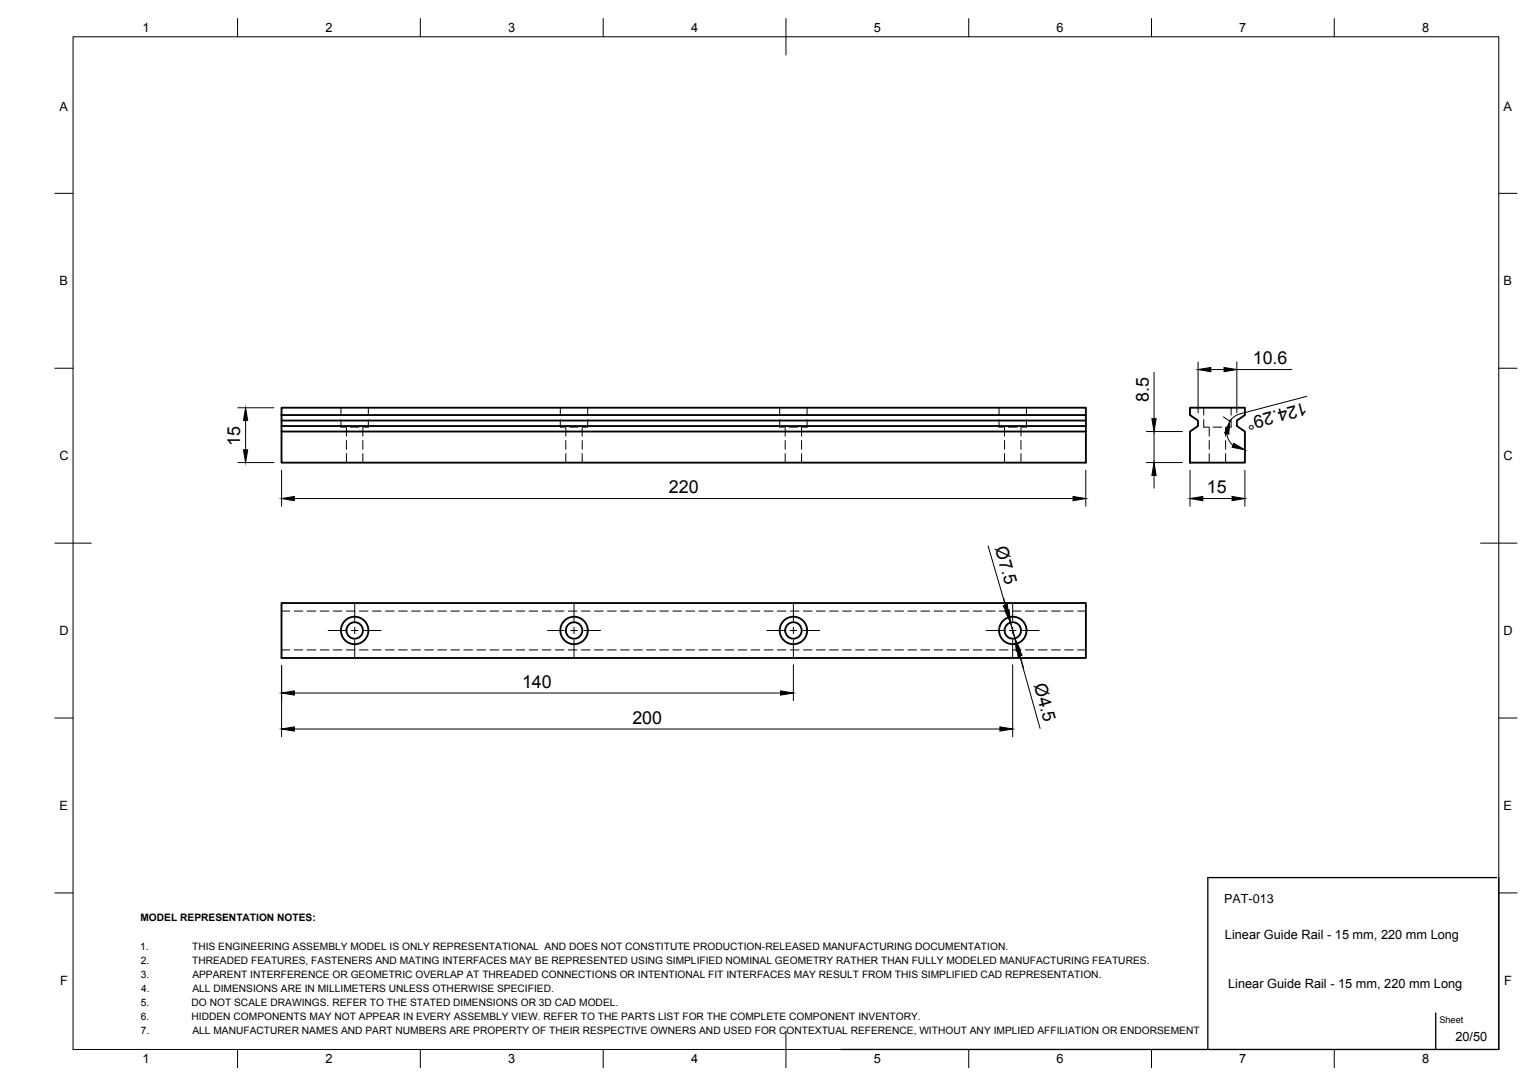
ISO-10303-21;
HEADER;
/* Generated by software containing ST-Developer
 * from STEP Tools, Inc. (www.steptools.com) 
 */

FILE_DESCRIPTION(
/* description */ ('Belt-driven linear axis on 2020 extrusion'),
/* implementation_level */ '2;1');

FILE_NAME(
/* name */ 'Linear Guide Rail - 15 mm, 220 mm Long.step',
/* time_stamp */ '2026-10-28T03:26:09-07:00',
/* author */ (''),
/* organization */ (''),
/* preprocessor_version */ 'ST-DEVELOPER v20.2',
/* originating_system */ 'Autodesk Translation Framework v15.17.0.0',
/* authorisation */ '');

FILE_SCHEMA (('AUTOMOTIVE_DESIGN { 1 0 10303 214 3 1 1 }'));
ENDSEC;

DATA;
#10=MECHANICAL_DESIGN_GEOMETRIC_PRESENTATION_REPRESENTATION('',(#642),#20096);
#540=SHAPE_REPRESENTATION_RELATIONSHIP('SRR','None',#20337,#586);
#586=ADVANCED_BREP_SHAPE_REPRESENTATION('',(#697),#20068);
#642=STYLED_ITEM('',(#20643),#697);
#697=MANIFOLD_SOLID_BREP('Body1',#10956);
#817=FACE_BOUND('',#2315,.T.);
#818=FACE_BOUND('',#2318,.T.);
#819=FACE_BOUND('',#2321,.T.);
#820=FACE_BOUND('',#2324,.T.);
#821=FACE_BOUND('',#2334,.T.);
#822=FACE_BOUND('',#2335,.T.);
#823=FACE_BOUND('',#2336,.T.);
#824=FACE_BOUND('',#2337,.T.);
#825=FACE_BOUND('',#2344,.T.);
#826=FACE_BOUND('',#2345,.T.);
#827=FACE_BOUND('',#2346,.T.);
#828=FACE_BOUND('',#2347,.T.);
#1092=PLANE('',#12149);
#1093=PLANE('',#12154);
#1094=PLANE('',#12159);
#1095=PLANE('',#12164);
#1096=PLANE('',#12174);
#1097=PLANE('',#12175);
#1098=PLANE('',#12176);
#1099=PLANE('',#12177);
#1100=PLANE('',#12178);
#1101=PLANE('',#12179);
#1102=PLANE('',#12180);
#1103=PLANE('',#12181);
#1104=PLANE('',#12182);
#1105=PLANE('',#12183);
#1106=PLANE('',#12184);
#1107=PLANE('',#12185);
#1108=PLANE('',#12186);
#1109=PLANE('',#12187);
#1592=FACE_OUTER_BOUND('',#2313,.T.);
#1593=FACE_OUTER_BOUND('',#2314,.T.);
#1594=FACE_OUTER_BOUND('',#2316,.T.);
#1595=FACE_OUTER_BOUND('',#2317,.T.);
#1596=FACE_OUTER_BOUND('',#2319,.T.);
#1597=FACE_OUTER_BOUND('',#2320,.T.);
#1598=FACE_OUTER_BOUND('',#2322,.T.);
#1599=FACE_OUTER_BOUND('',#2323,.T.);
#1600=FACE_OUTER_BOUND('',#2325,.T.);
#1601=FACE_OUTER_BOUND('',#2326,.T.);
#1602=FACE_OUTER_BOUND('',#2327,.T.);
#1603=FACE_OUTER_BOUND('',#2328,.T.);
#1604=FACE_OUTER_BOUND('',#2329,.T.);
#1605=FACE_OUTER_BOUND('',#2330,.T.);
#1606=FACE_OUTER_BOUND('',#2331,.T.);
#1607=FACE_OUTER_BOUND('',#2332,.T.);
#1608=FACE_OUTER_BOUND('',#2333,.T.);
#1609=FACE_OUTER_BOUND('',#2338,.T.);
#1610=FACE_OUTER_BOUND('',#2339,.T.);
#1611=FACE_OUTER_BOUND('',#2340,.T.);
#1612=FACE_OUTER_BOUND('',#2341,.T.);
#1613=FACE_OUTER_BOUND('',#2342,.T.);
#1614=FACE_OUTER_BOUND('',#2343,.T.);
#1615=FACE_OUTER_BOUND('',#2348,.T.);
#1616=FACE_OUTER_BOUND('',#2349,.T.);
#1617=FACE_OUTER_BOUND('',#2350,.T.);
#2313=EDGE_LOOP('',(#8845,#8846,#8847,#8848));
#2314=EDGE_LOOP('',(#8849));
#2315=EDGE_LOOP('',(#8850));
#2316=EDGE_LOOP('',(#8851,#8852,#8853,#8854));
#2317=EDGE_LOOP('',(#8855));
#2318=EDGE_LOOP('',(#8856));
#2319=EDGE_LOOP('',(#8857,#8858,#8859,#8860));
#2320=EDGE_LOOP('',(#8861));
#2321=EDGE_LOOP('',(#8862));
#2322=EDGE_LOOP('',(#8863,#8864,#8865,#8866));
#2323=EDGE_LOOP('',(#8867));
#2324=EDGE_LOOP('',(#8868));
#2325=EDGE_LOOP('',(#8869,#8870,#8871,#8872));
#2326=EDGE_LOOP('',(#8873,#8874,#8875,#8876));
#2327=EDGE_LOOP('',(#8877,#8878,#8879,#8880));
#2328=EDGE_LOOP('',(#8881,#8882,#8883,#8884));
#2329=EDGE_LOOP('',(#8885,#8886,#8887,#8888));
#2330=EDGE_LOOP('',(#8889,#8890,#8891,#8892));
#2331=EDGE_LOOP('',(#8893,#8894,#8895,#8896));
#2332=EDGE_LOOP('',(#8897,#8898,#8899,#8900));
#2333=EDGE_LOOP('',(#8901,#8902,#8903,#8904));
#2334=EDGE_LOOP('',(#8905));
#2335=EDGE_LOOP('',(#8906));
#2336=EDGE_LOOP('',(#8907));
#2337=EDGE_LOOP('',(#8908));
#2338=EDGE_LOOP('',(#8909,#8910,#8911,#8912));
#2339=EDGE_LOOP('',(#8913,#8914,#8915,#8916));
#2340=EDGE_LOOP('',(#8917,#8918,#8919,#8920));
#2341=EDGE_LOOP('',(#8921,#8922,#8923,#8924));
#2342=EDGE_LOOP('',(#8925,#8926,#8927,#8928));
#2343=EDGE_LOOP('',(#8929,#8930,#8931,#8932));
#2344=EDGE_LOOP('',(#8933));
#2345=EDGE_LOOP('',(#8934));
#2346=EDGE_LOOP('',(#8935));
#2347=EDGE_LOOP('',(#8936));
#2348=EDGE_LOOP('',(#8937,#8938,#8939,#8940));
#2349=EDGE_LOOP('',(#8941,#8942,#8943,#8944,#8945,#8946,#8947,#8948,#8949,
#8950,#8951,#8952));
#2350=EDGE_LOOP('',(#8953,#8954,#8955,#8956,#8957,#8958,#8959,#8960,#8961,
#8962,#8963,#8964));
#3160=LINE('',#18282,#4017);
#3161=LINE('',#18291,#4018);
#3162=LINE('',#18300,#4019);
#3163=LINE('',#18309,#4020);
#3164=LINE('',#18317,#4021);
#3165=LINE('',#18321,#4022);
#3166=LINE('',#18325,#4023);
#3167=LINE('',#18329,#4024);
#3168=LINE('',#18333,#4025);
#3169=LINE('',#18335,#4026);
#3170=LINE('',#18337,#4027);
#3171=LINE('',#18338,#4028);
#3172=LINE('',#18341,#4029);
#3173=LINE('',#18343,#4030);
#3174=LINE('',#18344,#4031);
#3175=LINE('',#18347,#4032);
#3176=LINE('',#18349,#4033);
#3177=LINE('',#18350,#4034);
#3178=LINE('',#18353,#4035);
#3179=LINE('',#18355,#4036);
#3180=LINE('',#18356,#4037);
#3181=LINE('',#18359,#4038);
#3182=LINE('',#18361,#4039);
#3183=LINE('',#18362,#4040);
#3184=LINE('',#18365,#4041);
#3185=LINE('',#18367,#4042);
#3186=LINE('',#18368,#4043);
#3187=LINE('',#18371,#4044);
#3188=LINE('',#18373,#4045);
#3189=LINE('',#18374,#4046);
#3190=LINE('',#18377,#4047);
#3191=LINE('',#18379,#4048);
#3192=LINE('',#18380,#4049);
#3193=LINE('',#18383,#4050);
#3194=LINE('',#18385,#4051);
#3195=LINE('',#18386,#4052);
#3196=LINE('',#18389,#4053);
#3197=LINE('',#18391,#4054);
#3198=LINE('',#18392,#4055);
#3199=LINE('',#18395,#4056);
#3200=LINE('',#18397,#4057);
#3201=LINE('',#18398,#4058);
#3202=LINE('',#18400,#4059);
#3203=LINE('',#18401,#4060);
#4017=VECTOR('',#14596,0.375);
#4018=VECTOR('',#14607,0.375);
#4019=VECTOR('',#14618,0.375);
#4020=VECTOR('',#14629,0.375);
#4021=VECTOR('',#14640,0.225);
#4022=VECTOR('',#14645,0.225);
#4023=VECTOR('',#14650,0.225);
#4024=VECTOR('',#14655,0.225000000000001);
#4025=VECTOR('',#14658,1.);
#4026=VECTOR('',#14659,1.);
#4027=VECTOR('',#14660,1.);
#4028=VECTOR('',#14661,1.);
#4029=VECTOR('',#14664,1.);
#4030=VECTOR('',#14665,1.);
#4031=VECTOR('',#14666,1.);
#4032=VECTOR('',#14669,1.);
#4033=VECTOR('',#14670,1.);
#4034=VECTOR('',#14671,1.);
#4035=VECTOR('',#14674,1.);
#4036=VECTOR('',#14675,1.);
#4037=VECTOR('',#14676,1.);
#4038=VECTOR('',#14679,1.);
#4039=VECTOR('',#14680,1.);
#4040=VECTOR('',#14681,1.);
#4041=VECTOR('',#14684,1.);
#4042=VECTOR('',#14685,1.);
#4043=VECTOR('',#14686,1.);
#4044=VECTOR('',#14689,1.);
#4045=VECTOR('',#14690,1.);
#4046=VECTOR('',#14691,1.);
#4047=VECTOR('',#14694,1.);
#4048=VECTOR('',#14695,1.);
#4049=VECTOR('',#14696,1.);
#4050=VECTOR('',#14699,1.);
#4051=VECTOR('',#14700,1.);
#4052=VECTOR('',#14701,1.);
#4053=VECTOR('',#14704,1.);
#4054=VECTOR('',#14705,1.);
#4055=VECTOR('',#14706,1.);
#4056=VECTOR('',#14709,1.);
#4057=VECTOR('',#14710,1.);
#4058=VECTOR('',#14711,1.);
#4059=VECTOR('',#14714,1.);
#4060=VECTOR('',#14715,1.);
#4660=CIRCLE('',#12147,0.375);
#4661=CIRCLE('',#12148,0.375);
#4662=CIRCLE('',#12150,0.225);
#4663=CIRCLE('',#12152,0.375);
#4664=CIRCLE('',#12153,0.375);
#4665=CIRCLE('',#12155,0.225);
#4666=CIRCLE('',#12157,0.375);
#4667=CIRCLE('',#12158,0.375);
#4668=CIRCLE('',#12160,0.225);
#4669=CIRCLE('',#12162,0.375);
#4670=CIRCLE('',#12163,0.375);
#4671=CIRCLE('',#12165,0.225000000000001);
#4672=CIRCLE('',#12167,0.225);
#4673=CIRCLE('',#12169,0.225);
#4674=CIRCLE('',#12171,0.225);
#4675=CIRCLE('',#12173,0.225000000000001);
#5431=VERTEX_POINT('',#18279);
#5432=VERTEX_POINT('',#18281);
#5433=VERTEX_POINT('',#18285);
#5434=VERTEX_POINT('',#18288);
#5435=VERTEX_POINT('',#18290);
#5436=VERTEX_POINT('',#18294);
#5437=VERTEX_POINT('',#18297);
#5438=VERTEX_POINT('',#18299);
#5439=VERTEX_POINT('',#18303);
#5440=VERTEX_POINT('',#18306);
#5441=VERTEX_POINT('',#18308);
#5442=VERTEX_POINT('',#18312);
#5443=VERTEX_POINT('',#18315);
#5444=VERTEX_POINT('',#18319);
#5445=VERTEX_POINT('',#18323);
#5446=VERTEX_POINT('',#18327);
#5447=VERTEX_POINT('',#18331);
#5448=VERTEX_POINT('',#18332);
#5449=VERTEX_POINT('',#18334);
#5450=VERTEX_POINT('',#18336);
#5451=VERTEX_POINT('',#18340);
#5452=VERTEX_POINT('',#18342);
#5453=VERTEX_POINT('',#18346);
#5454=VERTEX_POINT('',#18348);
#5455=VERTEX_POINT('',#18352);
#5456=VERTEX_POINT('',#18354);
#5457=VERTEX_POINT('',#18358);
#5458=VERTEX_POINT('',#18360);
#5459=VERTEX_POINT('',#18364);
#5460=VERTEX_POINT('',#18366);
#5461=VERTEX_POINT('',#18370);
#5462=VERTEX_POINT('',#18372);
#5463=VERTEX_POINT('',#18376);
#5464=VERTEX_POINT('',#18378);
#5465=VERTEX_POINT('',#18382);
#5466=VERTEX_POINT('',#18384);
#5467=VERTEX_POINT('',#18388);
#5468=VERTEX_POINT('',#18390);
#5469=VERTEX_POINT('',#18394);
#5470=VERTEX_POINT('',#18396);
#6637=EDGE_CURVE('',#5431,#5431,#4660,.T.);
#6638=EDGE_CURVE('',#5431,#5432,#3160,.T.);
#6639=EDGE_CURVE('',#5432,#5432,#4661,.T.);
#6640=EDGE_CURVE('',#5433,#5433,#4662,.T.);
#6641=EDGE_CURVE('',#5434,#5434,#4663,.T.);
#6642=EDGE_CURVE('',#5434,#5435,#3161,.T.);
#6643=EDGE_CURVE('',#5435,#5435,#4664,.T.);
#6644=EDGE_CURVE('',#5436,#5436,#4665,.T.);
#6645=EDGE_CURVE('',#5437,#5437,#4666,.T.);
#6646=EDGE_CURVE('',#5437,#5438,#3162,.T.);
#6647=EDGE_CURVE('',#5438,#5438,#4667,.T.);
#6648=EDGE_CURVE('',#5439,#5439,#4668,.T.);
#6649=EDGE_CURVE('',#5440,#5440,#4669,.T.);
#6650=EDGE_CURVE('',#5440,#5441,#3163,.T.);
#6651=EDGE_CURVE('',#5441,#5441,#4670,.T.);
#6652=EDGE_CURVE('',#5442,#5442,#4671,.T.);
#6653=EDGE_CURVE('',#5443,#5443,#4672,.T.);
#6654=EDGE_CURVE('',#5443,#5433,#3164,.T.);
#6655=EDGE_CURVE('',#5444,#5444,#4673,.T.);
#6656=EDGE_CURVE('',#5444,#5436,#3165,.T.);
#6657=EDGE_CURVE('',#5445,#5445,#4674,.T.);
#6658=EDGE_CURVE('',#5445,#5439,#3166,.T.);
#6659=EDGE_CURVE('',#5446,#5446,#4675,.T.);
#6660=EDGE_CURVE('',#5446,#5442,#3167,.T.);
#6661=EDGE_CURVE('',#5447,#5448,#3168,.T.);
#6662=EDGE_CURVE('',#5448,#5449,#3169,.T.);
#6663=EDGE_CURVE('',#5450,#5449,#3170,.T.);
#6664=EDGE_CURVE('',#5447,#5450,#3171,.T.);
#6665=EDGE_CURVE('',#5451,#5447,#3172,.T.);
#6666=EDGE_CURVE('',#5452,#5450,#3173,.T.);
#6667=EDGE_CURVE('',#5451,#5452,#3174,.T.);
#6668=EDGE_CURVE('',#5453,#5451,#3175,.T.);
#6669=EDGE_CURVE('',#5454,#5452,#3176,.T.);
#6670=EDGE_CURVE('',#5453,#5454,#3177,.T.);
#6671=EDGE_CURVE('',#5455,#5453,#3178,.T.);
#6672=EDGE_CURVE('',#5456,#5454,#3179,.T.);
#6673=EDGE_CURVE('',#5455,#5456,#3180,.T.);
#6674=EDGE_CURVE('',#5457,#5455,#3181,.T.);
#6675=EDGE_CURVE('',#5458,#5456,#3182,.T.);
#6676=EDGE_CURVE('',#5457,#5458,#3183,.T.);
#6677=EDGE_CURVE('',#5459,#5457,#3184,.T.);
#6678=EDGE_CURVE('',#5460,#5458,#3185,.T.);
#6679=EDGE_CURVE('',#5459,#5460,#3186,.T.);
#6680=EDGE_CURVE('',#5461,#5459,#3187,.T.);
#6681=EDGE_CURVE('',#5462,#5460,#3188,.T.);
#6682=EDGE_CURVE('',#5461,#5462,#3189,.T.);
#6683=EDGE_CURVE('',#5463,#5461,#3190,.T.);
#6684=EDGE_CURVE('',#5464,#5462,#3191,.T.);
#6685=EDGE_CURVE('',#5463,#5464,#3192,.T.);
#6686=EDGE_CURVE('',#5465,#5463,#3193,.T.);
#6687=EDGE_CURVE('',#5466,#5464,#3194,.T.);
#6688=EDGE_CURVE('',#5465,#5466,#3195,.T.);
#6689=EDGE_CURVE('',#5467,#5465,#3196,.T.);
#6690=EDGE_CURVE('',#5468,#5466,#3197,.T.);
#6691=EDGE_CURVE('',#5467,#5468,#3198,.T.);
#6692=EDGE_CURVE('',#5469,#5467,#3199,.T.);
#6693=EDGE_CURVE('',#5470,#5468,#3200,.T.);
#6694=EDGE_CURVE('',#5469,#5470,#3201,.T.);
#6695=EDGE_CURVE('',#5448,#5469,#3202,.T.);
#6696=EDGE_CURVE('',#5449,#5470,#3203,.T.);
#8845=ORIENTED_EDGE('',*,*,#6637,.F.);
#8846=ORIENTED_EDGE('',*,*,#6638,.T.);
#8847=ORIENTED_EDGE('',*,*,#6639,.F.);
#8848=ORIENTED_EDGE('',*,*,#6638,.F.);
#8849=ORIENTED_EDGE('',*,*,#6637,.T.);
#8850=ORIENTED_EDGE('',*,*,#6640,.F.);
#8851=ORIENTED_EDGE('',*,*,#6641,.F.);
#8852=ORIENTED_EDGE('',*,*,#6642,.T.);
#8853=ORIENTED_EDGE('',*,*,#6643,.F.);
#8854=ORIENTED_EDGE('',*,*,#6642,.F.);
#8855=ORIENTED_EDGE('',*,*,#6641,.T.);
#8856=ORIENTED_EDGE('',*,*,#6644,.F.);
#8857=ORIENTED_EDGE('',*,*,#6645,.F.);
#8858=ORIENTED_EDGE('',*,*,#6646,.T.);
#8859=ORIENTED_EDGE('',*,*,#6647,.F.);
#8860=ORIENTED_EDGE('',*,*,#6646,.F.);
#8861=ORIENTED_EDGE('',*,*,#6645,.T.);
#8862=ORIENTED_EDGE('',*,*,#6648,.F.);
#8863=ORIENTED_EDGE('',*,*,#6649,.F.);
#8864=ORIENTED_EDGE('',*,*,#6650,.T.);
#8865=ORIENTED_EDGE('',*,*,#6651,.F.);
#8866=ORIENTED_EDGE('',*,*,#6650,.F.);
#8867=ORIENTED_EDGE('',*,*,#6649,.T.);
#8868=ORIENTED_EDGE('',*,*,#6652,.F.);
#8869=ORIENTED_EDGE('',*,*,#6653,.F.);
#8870=ORIENTED_EDGE('',*,*,#6654,.T.);
#8871=ORIENTED_EDGE('',*,*,#6640,.T.);
#8872=ORIENTED_EDGE('',*,*,#6654,.F.);
#8873=ORIENTED_EDGE('',*,*,#6655,.F.);
#8874=ORIENTED_EDGE('',*,*,#6656,.T.);
#8875=ORIENTED_EDGE('',*,*,#6644,.T.);
#8876=ORIENTED_EDGE('',*,*,#6656,.F.);
#8877=ORIENTED_EDGE('',*,*,#6657,.F.);
#8878=ORIENTED_EDGE('',*,*,#6658,.T.);
#8879=ORIENTED_EDGE('',*,*,#6648,.T.);
#8880=ORIENTED_EDGE('',*,*,#6658,.F.);
#8881=ORIENTED_EDGE('',*,*,#6659,.F.);
#8882=ORIENTED_EDGE('',*,*,#6660,.T.);
#8883=ORIENTED_EDGE('',*,*,#6652,.T.);
#8884=ORIENTED_EDGE('',*,*,#6660,.F.);
#8885=ORIENTED_EDGE('',*,*,#6661,.T.);
#8886=ORIENTED_EDGE('',*,*,#6662,.T.);
#8887=ORIENTED_EDGE('',*,*,#6663,.F.);
#8888=ORIENTED_EDGE('',*,*,#6664,.F.);
#8889=ORIENTED_EDGE('',*,*,#6665,.T.);
#8890=ORIENTED_EDGE('',*,*,#6664,.T.);
#8891=ORIENTED_EDGE('',*,*,#6666,.F.);
#8892=ORIENTED_EDGE('',*,*,#6667,.F.);
#8893=ORIENTED_EDGE('',*,*,#6668,.T.);
#8894=ORIENTED_EDGE('',*,*,#6667,.T.);
#8895=ORIENTED_EDGE('',*,*,#6669,.F.);
#8896=ORIENTED_EDGE('',*,*,#6670,.F.);
#8897=ORIENTED_EDGE('',*,*,#6671,.T.);
#8898=ORIENTED_EDGE('',*,*,#6670,.T.);
#8899=ORIENTED_EDGE('',*,*,#6672,.F.);
#8900=ORIENTED_EDGE('',*,*,#6673,.F.);
#8901=ORIENTED_EDGE('',*,*,#6674,.T.);
#8902=ORIENTED_EDGE('',*,*,#6673,.T.);
#8903=ORIENTED_EDGE('',*,*,#6675,.F.);
#8904=ORIENTED_EDGE('',*,*,#6676,.F.);
#8905=ORIENTED_EDGE('',*,*,#6651,.T.);
#8906=ORIENTED_EDGE('',*,*,#6647,.T.);
#8907=ORIENTED_EDGE('',*,*,#6643,.T.);
#8908=ORIENTED_EDGE('',*,*,#6639,.T.);
#8909=ORIENTED_EDGE('',*,*,#6677,.T.);
#8910=ORIENTED_EDGE('',*,*,#6676,.T.);
#8911=ORIENTED_EDGE('',*,*,#6678,.F.);
#8912=ORIENTED_EDGE('',*,*,#6679,.F.);
#8913=ORIENTED_EDGE('',*,*,#6680,.T.);
#8914=ORIENTED_EDGE('',*,*,#6679,.T.);
#8915=ORIENTED_EDGE('',*,*,#6681,.F.);
#8916=ORIENTED_EDGE('',*,*,#6682,.F.);
#8917=ORIENTED_EDGE('',*,*,#6683,.T.);
#8918=ORIENTED_EDGE('',*,*,#6682,.T.);
#8919=ORIENTED_EDGE('',*,*,#6684,.F.);
#8920=ORIENTED_EDGE('',*,*,#6685,.F.);
#8921=ORIENTED_EDGE('',*,*,#6686,.T.);
#8922=ORIENTED_EDGE('',*,*,#6685,.T.);
#8923=ORIENTED_EDGE('',*,*,#6687,.F.);
#8924=ORIENTED_EDGE('',*,*,#6688,.F.);
#8925=ORIENTED_EDGE('',*,*,#6689,.T.);
#8926=ORIENTED_EDGE('',*,*,#6688,.T.);
#8927=ORIENTED_EDGE('',*,*,#6690,.F.);
#8928=ORIENTED_EDGE('',*,*,#6691,.F.);
#8929=ORIENTED_EDGE('',*,*,#6692,.T.);
#8930=ORIENTED_EDGE('',*,*,#6691,.T.);
#8931=ORIENTED_EDGE('',*,*,#6693,.F.);
#8932=ORIENTED_EDGE('',*,*,#6694,.F.);
#8933=ORIENTED_EDGE('',*,*,#6653,.T.);
#8934=ORIENTED_EDGE('',*,*,#6655,.T.);
#8935=ORIENTED_EDGE('',*,*,#6657,.T.);
#8936=ORIENTED_EDGE('',*,*,#6659,.T.);
#8937=ORIENTED_EDGE('',*,*,#6695,.T.);
#8938=ORIENTED_EDGE('',*,*,#6694,.T.);
#8939=ORIENTED_EDGE('',*,*,#6696,.F.);
#8940=ORIENTED_EDGE('',*,*,#6662,.F.);
#8941=ORIENTED_EDGE('',*,*,#6696,.T.);
#8942=ORIENTED_EDGE('',*,*,#6693,.T.);
#8943=ORIENTED_EDGE('',*,*,#6690,.T.);
#8944=ORIENTED_EDGE('',*,*,#6687,.T.);
#8945=ORIENTED_EDGE('',*,*,#6684,.T.);
#8946=ORIENTED_EDGE('',*,*,#6681,.T.);
#8947=ORIENTED_EDGE('',*,*,#6678,.T.);
#8948=ORIENTED_EDGE('',*,*,#6675,.T.);
#8949=ORIENTED_EDGE('',*,*,#6672,.T.);
#8950=ORIENTED_EDGE('',*,*,#6669,.T.);
#8951=ORIENTED_EDGE('',*,*,#6666,.T.);
#8952=ORIENTED_EDGE('',*,*,#6663,.T.);
#8953=ORIENTED_EDGE('',*,*,#6695,.F.);
#8954=ORIENTED_EDGE('',*,*,#6661,.F.);
#8955=ORIENTED_EDGE('',*,*,#6665,.F.);
#8956=ORIENTED_EDGE('',*,*,#6668,.F.);
#8957=ORIENTED_EDGE('',*,*,#6671,.F.);
#8958=ORIENTED_EDGE('',*,*,#6674,.F.);
#8959=ORIENTED_EDGE('',*,*,#6677,.F.);
#8960=ORIENTED_EDGE('',*,*,#6680,.F.);
#8961=ORIENTED_EDGE('',*,*,#6683,.F.);
#8962=ORIENTED_EDGE('',*,*,#6686,.F.);
#8963=ORIENTED_EDGE('',*,*,#6689,.F.);
#8964=ORIENTED_EDGE('',*,*,#6692,.F.);
#10191=CYLINDRICAL_SURFACE('',#12146,0.375);
#10192=CYLINDRICAL_SURFACE('',#12151,0.375);
#10193=CYLINDRICAL_SURFACE('',#12156,0.375);
#10194=CYLINDRICAL_SURFACE('',#12161,0.375);
#10195=CYLINDRICAL_SURFACE('',#12166,0.225);
#10196=CYLINDRICAL_SURFACE('',#12168,0.225);
#10197=CYLINDRICAL_SURFACE('',#12170,0.225);
#10198=CYLINDRICAL_SURFACE('',#12172,0.225000000000001);
#10643=ADVANCED_FACE('',(#1592),#10191,.F.);
#10644=ADVANCED_FACE('',(#1593,#817),#1092,.T.);
#10645=ADVANCED_FACE('',(#1594),#10192,.F.);
#10646=ADVANCED_FACE('',(#1595,#818),#1093,.T.);
#10647=ADVANCED_FACE('',(#1596),#10193,.F.);
#10648=ADVANCED_FACE('',(#1597,#819),#1094,.T.);
#10649=ADVANCED_FACE('',(#1598),#10194,.F.);
#10650=ADVANCED_FACE('',(#1599,#820),#1095,.T.);
#10651=ADVANCED_FACE('',(#1600),#10195,.F.);
#10652=ADVANCED_FACE('',(#1601),#10196,.F.);
#10653=ADVANCED_FACE('',(#1602),#10197,.F.);
#10654=ADVANCED_FACE('',(#1603),#10198,.F.);
#10655=ADVANCED_FACE('',(#1604),#1096,.T.);
#10656=ADVANCED_FACE('',(#1605),#1097,.T.);
#10657=ADVANCED_FACE('',(#1606),#1098,.T.);
#10658=ADVANCED_FACE('',(#1607),#1099,.T.);
#10659=ADVANCED_FACE('',(#1608,#821,#822,#823,#824),#1100,.T.);
#10660=ADVANCED_FACE('',(#1609),#1101,.T.);
#10661=ADVANCED_FACE('',(#1610),#1102,.T.);
#10662=ADVANCED_FACE('',(#1611),#1103,.T.);
#10663=ADVANCED_FACE('',(#1612),#1104,.T.);
#10664=ADVANCED_FACE('',(#1613),#1105,.T.);
#10665=ADVANCED_FACE('',(#1614,#825,#826,#827,#828),#1106,.T.);
#10666=ADVANCED_FACE('',(#1615),#1107,.T.);
#10667=ADVANCED_FACE('',(#1616),#1108,.T.);
#10668=ADVANCED_FACE('',(#1617),#1109,.F.);
#10956=CLOSED_SHELL('',(#10643,#10644,#10645,#10646,#10647,#10648,#10649,
#10650,#10651,#10652,#10653,#10654,#10655,#10656,#10657,#10658,#10659,#10660,
#10661,#10662,#10663,#10664,#10665,#10666,#10667,#10668));
#12145=AXIS2_PLACEMENT_3D('',#18277,#14590,#14591);
#12146=AXIS2_PLACEMENT_3D('',#18278,#14592,#14593);
#12147=AXIS2_PLACEMENT_3D('',#18280,#14594,#14595);
#12148=AXIS2_PLACEMENT_3D('',#18283,#14597,#14598);
#12149=AXIS2_PLACEMENT_3D('',#18284,#14599,#14600);
#12150=AXIS2_PLACEMENT_3D('',#18286,#14601,#14602);
#12151=AXIS2_PLACEMENT_3D('',#18287,#14603,#14604);
#12152=AXIS2_PLACEMENT_3D('',#18289,#14605,#14606);
#12153=AXIS2_PLACEMENT_3D('',#18292,#14608,#14609);
#12154=AXIS2_PLACEMENT_3D('',#18293,#14610,#14611);
#12155=AXIS2_PLACEMENT_3D('',#18295,#14612,#14613);
#12156=AXIS2_PLACEMENT_3D('',#18296,#14614,#14615);
#12157=AXIS2_PLACEMENT_3D('',#18298,#14616,#14617);
#12158=AXIS2_PLACEMENT_3D('',#18301,#14619,#14620);
#12159=AXIS2_PLACEMENT_3D('',#18302,#14621,#14622);
#12160=AXIS2_PLACEMENT_3D('',#18304,#14623,#14624);
#12161=AXIS2_PLACEMENT_3D('',#18305,#14625,#14626);
#12162=AXIS2_PLACEMENT_3D('',#18307,#14627,#14628);
#12163=AXIS2_PLACEMENT_3D('',#18310,#14630,#14631);
#12164=AXIS2_PLACEMENT_3D('',#18311,#14632,#14633);
#12165=AXIS2_PLACEMENT_3D('',#18313,#14634,#14635);
#12166=AXIS2_PLACEMENT_3D('',#18314,#14636,#14637);
#12167=AXIS2_PLACEMENT_3D('',#18316,#14638,#14639);
#12168=AXIS2_PLACEMENT_3D('',#18318,#14641,#14642);
#12169=AXIS2_PLACEMENT_3D('',#18320,#14643,#14644);
#12170=AXIS2_PLACEMENT_3D('',#18322,#14646,#14647);
#12171=AXIS2_PLACEMENT_3D('',#18324,#14648,#14649);
#12172=AXIS2_PLACEMENT_3D('',#18326,#14651,#14652);
#12173=AXIS2_PLACEMENT_3D('',#18328,#14653,#14654);
#12174=AXIS2_PLACEMENT_3D('',#18330,#14656,#14657);
#12175=AXIS2_PLACEMENT_3D('',#18339,#14662,#14663);
#12176=AXIS2_PLACEMENT_3D('',#18345,#14667,#14668);
#12177=AXIS2_PLACEMENT_3D('',#18351,#14672,#14673);
#12178=AXIS2_PLACEMENT_3D('',#18357,#14677,#14678);
#12179=AXIS2_PLACEMENT_3D('',#18363,#14682,#14683);
#12180=AXIS2_PLACEMENT_3D('',#18369,#14687,#14688);
#12181=AXIS2_PLACEMENT_3D('',#18375,#14692,#14693);
#12182=AXIS2_PLACEMENT_3D('',#18381,#14697,#14698);
#12183=AXIS2_PLACEMENT_3D('',#18387,#14702,#14703);
#12184=AXIS2_PLACEMENT_3D('',#18393,#14707,#14708);
#12185=AXIS2_PLACEMENT_3D('',#18399,#14712,#14713);
#12186=AXIS2_PLACEMENT_3D('',#18402,#14716,#14717);
#12187=AXIS2_PLACEMENT_3D('',#18403,#14718,#14719);
#14590=DIRECTION('axis',(0.,0.,1.));
#14591=DIRECTION('refdir',(1.,0.,0.));
#14592=DIRECTION('center_axis',(0.,0.,1.));
#14593=DIRECTION('ref_axis',(1.,0.,0.));
#14594=DIRECTION('center_axis',(0.,0.,1.));
#14595=DIRECTION('ref_axis',(1.,0.,0.));
#14596=DIRECTION('',(0.,0.,1.));
#14597=DIRECTION('center_axis',(0.,0.,-1.));
#14598=DIRECTION('ref_axis',(1.,0.,0.));
#14599=DIRECTION('center_axis',(0.,0.,1.));
#14600=DIRECTION('ref_axis',(1.,0.,0.));
#14601=DIRECTION('center_axis',(0.,0.,1.));
#14602=DIRECTION('ref_axis',(1.,0.,0.));
#14603=DIRECTION('center_axis',(0.,0.,1.));
#14604=DIRECTION('ref_axis',(1.,0.,0.));
#14605=DIRECTION('center_axis',(0.,0.,1.));
#14606=DIRECTION('ref_axis',(1.,0.,0.));
#14607=DIRECTION('',(0.,0.,1.));
#14608=DIRECTION('center_axis',(0.,0.,-1.));
#14609=DIRECTION('ref_axis',(1.,0.,0.));
#14610=DIRECTION('center_axis',(0.,0.,1.));
#14611=DIRECTION('ref_axis',(1.,0.,0.));
#14612=DIRECTION('center_axis',(0.,0.,1.));
#14613=DIRECTION('ref_axis',(1.,0.,0.));
#14614=DIRECTION('center_axis',(0.,0.,1.));
#14615=DIRECTION('ref_axis',(1.,0.,0.));
#14616=DIRECTION('center_axis',(0.,0.,1.));
#14617=DIRECTION('ref_axis',(1.,0.,0.));
#14618=DIRECTION('',(0.,0.,1.));
#14619=DIRECTION('center_axis',(0.,0.,-1.));
#14620=DIRECTION('ref_axis',(1.,0.,0.));
#14621=DIRECTION('center_axis',(0.,0.,1.));
#14622=DIRECTION('ref_axis',(1.,0.,0.));
#14623=DIRECTION('center_axis',(0.,0.,1.));
#14624=DIRECTION('ref_axis',(1.,0.,0.));
#14625=DIRECTION('center_axis',(0.,0.,1.));
#14626=DIRECTION('ref_axis',(1.,0.,0.));
#14627=DIRECTION('center_axis',(0.,0.,1.));
#14628=DIRECTION('ref_axis',(1.,0.,0.));
#14629=DIRECTION('',(0.,0.,1.));
#14630=DIRECTION('center_axis',(0.,0.,-1.));
#14631=DIRECTION('ref_axis',(1.,0.,0.));
#14632=DIRECTION('center_axis',(0.,0.,1.));
#14633=DIRECTION('ref_axis',(1.,0.,0.));
#14634=DIRECTION('center_axis',(0.,0.,1.));
#14635=DIRECTION('ref_axis',(1.,0.,0.));
#14636=DIRECTION('center_axis',(0.,0.,1.));
#14637=DIRECTION('ref_axis',(1.,0.,0.));
#14638=DIRECTION('center_axis',(0.,0.,1.));
#14639=DIRECTION('ref_axis',(1.,0.,0.));
#14640=DIRECTION('',(0.,0.,1.));
#14641=DIRECTION('center_axis',(0.,0.,1.));
#14642=DIRECTION('ref_axis',(1.,0.,0.));
#14643=DIRECTION('center_axis',(0.,0.,1.));
#14644=DIRECTION('ref_axis',(1.,0.,0.));
#14645=DIRECTION('',(0.,0.,1.));
#14646=DIRECTION('center_axis',(0.,0.,1.));
#14647=DIRECTION('ref_axis',(1.,0.,0.));
#14648=DIRECTION('center_axis',(0.,0.,1.));
#14649=DIRECTION('ref_axis',(1.,0.,0.));
#14650=DIRECTION('',(0.,0.,1.));
#14651=DIRECTION('center_axis',(0.,0.,1.));
#14652=DIRECTION('ref_axis',(1.,0.,0.));
#14653=DIRECTION('center_axis',(0.,0.,1.));
#14654=DIRECTION('ref_axis',(1.,0.,0.));
#14655=DIRECTION('',(0.,0.,1.));
#14656=DIRECTION('center_axis',(0.,-0.56333682464151,0.826227342807548));
#14657=DIRECTION('ref_axis',(0.,-0.826227342807548,-0.56333682464151));
#14658=DIRECTION('',(0.,-0.826227342807548,-0.56333682464151));
#14659=DIRECTION('',(1.,0.,0.));
#14660=DIRECTION('',(0.,-0.826227342807548,-0.56333682464151));
#14661=DIRECTION('',(1.,0.,0.));
#14662=DIRECTION('center_axis',(0.,-1.,0.));
#14663=DIRECTION('ref_axis',(0.,0.,-1.));
#14664=DIRECTION('',(0.,0.,-1.));
#14665=DIRECTION('',(0.,0.,-1.));
#14666=DIRECTION('',(1.,0.,0.));
#14667=DIRECTION('center_axis',(0.,-0.56333682464151,-0.826227342807548));
#14668=DIRECTION('ref_axis',(0.,0.826227342807548,-0.56333682464151));
#14669=DIRECTION('',(0.,0.826227342807548,-0.56333682464151));
#14670=DIRECTION('',(0.,0.826227342807548,-0.56333682464151));
#14671=DIRECTION('',(1.,0.,0.));
#14672=DIRECTION('center_axis',(0.,-1.,0.));
#14673=DIRECTION('ref_axis',(0.,0.,-1.));
#14674=DIRECTION('',(0.,0.,-1.));
#14675=DIRECTION('',(0.,0.,-1.));
#14676=DIRECTION('',(1.,0.,0.));
#14677=DIRECTION('center_axis',(0.,0.,1.));
#14678=DIRECTION('ref_axis',(0.,-1.,0.));
#14679=DIRECTION('',(0.,-1.,0.));
#14680=DIRECTION('',(0.,-1.,0.));
#14681=DIRECTION('',(1.,0.,0.));
#14682=DIRECTION('center_axis',(0.,1.,0.));
#14683=DIRECTION('ref_axis',(0.,0.,1.));
#14684=DIRECTION('',(0.,0.,1.));
#14685=DIRECTION('',(0.,0.,1.));
#14686=DIRECTION('',(1.,0.,0.));
#14687=DIRECTION('center_axis',(0.,0.56333682464151,-0.826227342807548));
#14688=DIRECTION('ref_axis',(0.,0.826227342807548,0.56333682464151));
#14689=DIRECTION('',(0.,0.826227342807548,0.56333682464151));
#14690=DIRECTION('',(0.,0.826227342807548,0.56333682464151));
#14691=DIRECTION('',(1.,0.,0.));
#14692=DIRECTION('center_axis',(0.,1.,0.));
#14693=DIRECTION('ref_axis',(0.,0.,1.));
#14694=DIRECTION('',(0.,0.,1.));
#14695=DIRECTION('',(0.,0.,1.));
#14696=DIRECTION('',(1.,0.,0.));
#14697=DIRECTION('center_axis',(0.,0.56333682464151,0.826227342807548));
#14698=DIRECTION('ref_axis',(0.,-0.826227342807548,0.56333682464151));
#14699=DIRECTION('',(0.,-0.826227342807548,0.56333682464151));
#14700=DIRECTION('',(0.,-0.826227342807548,0.56333682464151));
#14701=DIRECTION('',(1.,0.,0.));
#14702=DIRECTION('center_axis',(0.,1.,0.));
#14703=DIRECTION('ref_axis',(0.,0.,1.));
#14704=DIRECTION('',(0.,0.,1.));
#14705=DIRECTION('',(0.,0.,1.));
#14706=DIRECTION('',(1.,0.,0.));
#14707=DIRECTION('center_axis',(0.,0.,-1.));
#14708=DIRECTION('ref_axis',(0.,1.,0.));
#14709=DIRECTION('',(0.,1.,0.));
#14710=DIRECTION('',(0.,1.,0.));
#14711=DIRECTION('',(1.,0.,0.));
#14712=DIRECTION('center_axis',(0.,-1.,0.));
#14713=DIRECTION('ref_axis',(0.,0.,-1.));
#14714=DIRECTION('',(0.,0.,-1.));
#14715=DIRECTION('',(0.,0.,-1.));
#14716=DIRECTION('center_axis',(1.,0.,0.));
#14717=DIRECTION('ref_axis',(0.,0.,-1.));
#14718=DIRECTION('center_axis',(1.,0.,0.));
#14719=DIRECTION('ref_axis',(0.,0.,-1.));
#18277=CARTESIAN_POINT('',(0.,0.,0.));
#18278=CARTESIAN_POINT('Origin',(14.,0.,0.97));
#18279=CARTESIAN_POINT('',(13.625,-4.59242549680257E-17,0.97));
#18280=CARTESIAN_POINT('Origin',(14.,0.,0.97));
#18281=CARTESIAN_POINT('',(13.625,4.59242549680257E-17,1.5));
#18282=CARTESIAN_POINT('',(13.625,-4.59242549680257E-17,0.97));
#18283=CARTESIAN_POINT('Origin',(14.,0.,1.5));
#18284=CARTESIAN_POINT('Origin',(14.,0.,0.97));
#18285=CARTESIAN_POINT('',(13.775,-2.75545529808154E-17,0.97));
#18286=CARTESIAN_POINT('Origin',(14.,0.,0.97));
#18287=CARTESIAN_POINT('Origin',(8.,0.,0.97));
#18288=CARTESIAN_POINT('',(7.625,-4.59242549680257E-17,0.97));
#18289=CARTESIAN_POINT('Origin',(8.,0.,0.97));
#18290=CARTESIAN_POINT('',(7.625,4.59242549680257E-17,1.5));
#18291=CARTESIAN_POINT('',(7.625,-4.59242549680257E-17,0.97));
#18292=CARTESIAN_POINT('Origin',(8.,0.,1.5));
#18293=CARTESIAN_POINT('Origin',(8.,0.,0.97));
#18294=CARTESIAN_POINT('',(7.775,-2.75545529808154E-17,0.97));
#18295=CARTESIAN_POINT('Origin',(8.,0.,0.97));
#18296=CARTESIAN_POINT('Origin',(2.,0.,0.97));
#18297=CARTESIAN_POINT('',(1.625,-4.59242549680257E-17,0.97));
#18298=CARTESIAN_POINT('Origin',(2.,0.,0.97));
#18299=CARTESIAN_POINT('',(1.625,4.59242549680257E-17,1.5));
#18300=CARTESIAN_POINT('',(1.625,-4.59242549680257E-17,0.97));
#18301=CARTESIAN_POINT('Origin',(2.,0.,1.5));
#18302=CARTESIAN_POINT('Origin',(2.,0.,0.97));
#18303=CARTESIAN_POINT('',(1.775,-2.75545529808155E-17,0.97));
#18304=CARTESIAN_POINT('Origin',(2.,0.,0.97));
#18305=CARTESIAN_POINT('Origin',(20.,0.,0.97));
#18306=CARTESIAN_POINT('',(19.625,-4.59242549680257E-17,0.97));
#18307=CARTESIAN_POINT('Origin',(20.,0.,0.97));
#18308=CARTESIAN_POINT('',(19.625,4.59242549680257E-17,1.5));
#18309=CARTESIAN_POINT('',(19.625,-4.59242549680257E-17,0.97));
#18310=CARTESIAN_POINT('Origin',(20.,0.,1.5));
#18311=CARTESIAN_POINT('Origin',(20.,0.,0.97));
#18312=CARTESIAN_POINT('',(19.775,-2.75545529808156E-17,0.97));
#18313=CARTESIAN_POINT('Origin',(20.,0.,0.97));
#18314=CARTESIAN_POINT('Origin',(14.,0.,-0.1));
#18315=CARTESIAN_POINT('',(13.775,-2.75545529808154E-17,0.));
#18316=CARTESIAN_POINT('Origin',(14.,0.,0.));
#18317=CARTESIAN_POINT('',(13.775,-2.75545529808154E-17,-0.1));
#18318=CARTESIAN_POINT('Origin',(8.,0.,-0.1));
#18319=CARTESIAN_POINT('',(7.775,-2.75545529808154E-17,0.));
#18320=CARTESIAN_POINT('Origin',(8.,0.,0.));
#18321=CARTESIAN_POINT('',(7.775,-2.75545529808154E-17,-0.1));
#18322=CARTESIAN_POINT('Origin',(2.,0.,-0.1));
#18323=CARTESIAN_POINT('',(1.775,-2.75545529808155E-17,0.));
#18324=CARTESIAN_POINT('Origin',(2.,0.,0.));
#18325=CARTESIAN_POINT('',(1.775,-2.75545529808155E-17,-0.1));
#18326=CARTESIAN_POINT('Origin',(20.,0.,-0.1));
#18327=CARTESIAN_POINT('',(19.775,-2.75545529808156E-17,0.));
#18328=CARTESIAN_POINT('Origin',(20.,0.,0.));
#18329=CARTESIAN_POINT('',(19.775,-2.75545529808156E-17,-0.1));
#18330=CARTESIAN_POINT('Origin',(0.,-0.53,1.));
#18331=CARTESIAN_POINT('',(0.,-0.53,1.));
#18332=CARTESIAN_POINT('',(0.,-0.75,0.85));
#18333=CARTESIAN_POINT('',(0.,-0.53,1.));
#18334=CARTESIAN_POINT('',(22.,-0.75,0.85));
#18335=CARTESIAN_POINT('',(0.,-0.75,0.85));
#18336=CARTESIAN_POINT('',(22.,-0.53,1.));
#18337=CARTESIAN_POINT('',(22.,-0.53,1.));
#18338=CARTESIAN_POINT('',(0.,-0.53,1.));
#18339=CARTESIAN_POINT('Origin',(0.,-0.53,1.15));
#18340=CARTESIAN_POINT('',(0.,-0.53,1.15));
#18341=CARTESIAN_POINT('',(0.,-0.53,1.15));
#18342=CARTESIAN_POINT('',(22.,-0.53,1.15));
#18343=CARTESIAN_POINT('',(22.,-0.53,1.15));
#18344=CARTESIAN_POINT('',(0.,-0.53,1.15));
#18345=CARTESIAN_POINT('Origin',(0.,-0.75,1.3));
#18346=CARTESIAN_POINT('',(0.,-0.75,1.3));
#18347=CARTESIAN_POINT('',(0.,-0.75,1.3));
#18348=CARTESIAN_POINT('',(22.,-0.75,1.3));
#18349=CARTESIAN_POINT('',(22.,-0.75,1.3));
#18350=CARTESIAN_POINT('',(0.,-0.75,1.3));
#18351=CARTESIAN_POINT('Origin',(0.,-0.75,1.5));
#18352=CARTESIAN_POINT('',(0.,-0.75,1.5));
#18353=CARTESIAN_POINT('',(0.,-0.75,1.5));
#18354=CARTESIAN_POINT('',(22.,-0.75,1.5));
#18355=CARTESIAN_POINT('',(22.,-0.75,1.5));
#18356=CARTESIAN_POINT('',(0.,-0.75,1.5));
#18357=CARTESIAN_POINT('Origin',(0.,0.75,1.5));
#18358=CARTESIAN_POINT('',(0.,0.75,1.5));
#18359=CARTESIAN_POINT('',(0.,0.75,1.5));
#18360=CARTESIAN_POINT('',(22.,0.75,1.5));
#18361=CARTESIAN_POINT('',(22.,0.75,1.5));
#18362=CARTESIAN_POINT('',(0.,0.75,1.5));
#18363=CARTESIAN_POINT('Origin',(0.,0.75,1.3));
#18364=CARTESIAN_POINT('',(0.,0.75,1.3));
#18365=CARTESIAN_POINT('',(0.,0.75,1.3));
#18366=CARTESIAN_POINT('',(22.,0.75,1.3));
#18367=CARTESIAN_POINT('',(22.,0.75,1.3));
#18368=CARTESIAN_POINT('',(0.,0.75,1.3));
#18369=CARTESIAN_POINT('Origin',(0.,0.53,1.15));
#18370=CARTESIAN_POINT('',(0.,0.53,1.15));
#18371=CARTESIAN_POINT('',(0.,0.53,1.15));
#18372=CARTESIAN_POINT('',(22.,0.53,1.15));
#18373=CARTESIAN_POINT('',(22.,0.53,1.15));
#18374=CARTESIAN_POINT('',(0.,0.53,1.15));
#18375=CARTESIAN_POINT('Origin',(0.,0.53,1.));
#18376=CARTESIAN_POINT('',(0.,0.53,1.));
#18377=CARTESIAN_POINT('',(0.,0.53,1.));
#18378=CARTESIAN_POINT('',(22.,0.53,1.));
#18379=CARTESIAN_POINT('',(22.,0.53,1.));
#18380=CARTESIAN_POINT('',(0.,0.53,1.));
#18381=CARTESIAN_POINT('Origin',(0.,0.75,0.85));
#18382=CARTESIAN_POINT('',(0.,0.75,0.85));
#18383=CARTESIAN_POINT('',(0.,0.75,0.85));
#18384=CARTESIAN_POINT('',(22.,0.75,0.85));
#18385=CARTESIAN_POINT('',(22.,0.75,0.85));
#18386=CARTESIAN_POINT('',(0.,0.75,0.85));
#18387=CARTESIAN_POINT('Origin',(0.,0.75,0.));
#18388=CARTESIAN_POINT('',(0.,0.75,0.));
#18389=CARTESIAN_POINT('',(0.,0.75,0.));
#18390=CARTESIAN_POINT('',(22.,0.75,0.));
#18391=CARTESIAN_POINT('',(22.,0.75,0.));
#18392=CARTESIAN_POINT('',(0.,0.75,0.));
#18393=CARTESIAN_POINT('Origin',(0.,-0.75,0.));
#18394=CARTESIAN_POINT('',(0.,-0.75,0.));
#18395=CARTESIAN_POINT('',(0.,-0.75,0.));
#18396=CARTESIAN_POINT('',(22.,-0.75,0.));
#18397=CARTESIAN_POINT('',(22.,-0.75,0.));
#18398=CARTESIAN_POINT('',(0.,-0.75,0.));
#18399=CARTESIAN_POINT('Origin',(0.,-0.75,0.85));
#18400=CARTESIAN_POINT('',(0.,-0.75,0.85));
#18401=CARTESIAN_POINT('',(22.,-0.75,0.85));
#18402=CARTESIAN_POINT('Origin',(22.,0.,0.75));
#18403=CARTESIAN_POINT('Origin',(0.,0.,0.75));
#20014=UNCERTAINTY_MEASURE_WITH_UNIT(LENGTH_MEASURE(0.001),#20097,
'DISTANCE_ACCURACY_VALUE',
'Maximum model space distance between geometric entities at asserted c
onnectivities');
#20042=UNCERTAINTY_MEASURE_WITH_UNIT(LENGTH_MEASURE(0.001),#20097,
'DISTANCE_ACCURACY_VALUE',
'Maximum model space distance between geometric entities at asserted c
onnectivities');
#20068=(
GEOMETRIC_REPRESENTATION_CONTEXT(3)
GLOBAL_UNCERTAINTY_ASSIGNED_CONTEXT((#20014))
GLOBAL_UNIT_ASSIGNED_CONTEXT((#20097,#20099,#20100))
REPRESENTATION_CONTEXT('','3D')
);
#20096=(
GEOMETRIC_REPRESENTATION_CONTEXT(3)
GLOBAL_UNCERTAINTY_ASSIGNED_CONTEXT((#20042))
GLOBAL_UNIT_ASSIGNED_CONTEXT((#20097,#20099,#20100))
REPRESENTATION_CONTEXT('','3D')
);
#20097=(
LENGTH_UNIT()
NAMED_UNIT(*)
SI_UNIT(.CENTI.,.METRE.)
);
#20099=(
NAMED_UNIT(*)
PLANE_ANGLE_UNIT()
SI_UNIT($,.RADIAN.)
);
#20100=(
NAMED_UNIT(*)
SI_UNIT($,.STERADIAN.)
SOLID_ANGLE_UNIT()
);
#20126=SHAPE_DEFINITION_REPRESENTATION(#20184,#20337);
#20184=PRODUCT_DEFINITION_SHAPE('',$,#20391);
#20337=SHAPE_REPRESENTATION('',(#12145),#20068);
#20365=PRODUCT_DEFINITION_CONTEXT('part definition',#20526,'design');
#20391=PRODUCT_DEFINITION('Linear Guide Rail - 15 mm, 220 mm Long',
'Linear Guide Rail - 15 mm, 220 mm Long',#20444,#20365);
#20444=PRODUCT_DEFINITION_FORMATION('',$,#20553);
#20526=APPLICATION_CONTEXT(
'Core Data for Automotive Mechanical Design Process');
#20527=PRODUCT_CONTEXT('part definition',#20526,'mechanical');
#20553=PRODUCT('Linear Guide Rail - 15 mm, 220 mm Long',
'Linear Guide Rail - 15 mm, 220 mm Long',
'Linear Guide Rail - 15 mm, 220 mm Long',(#20527));
#20637=COLOUR_RGB('Sky Blue',0.24,0.69,0.87);
#20638=FILL_AREA_STYLE_COLOUR('',#20637);
#20639=FILL_AREA_STYLE('',(#20638));
#20640=SURFACE_STYLE_FILL_AREA(#20639);
#20641=SURFACE_SIDE_STYLE('',(#20640));
#20642=SURFACE_STYLE_USAGE(.BOTH.,#20641);
#20643=PRESENTATION_STYLE_ASSIGNMENT((#20642));
ENDSEC;
END-ISO-10303-21;
